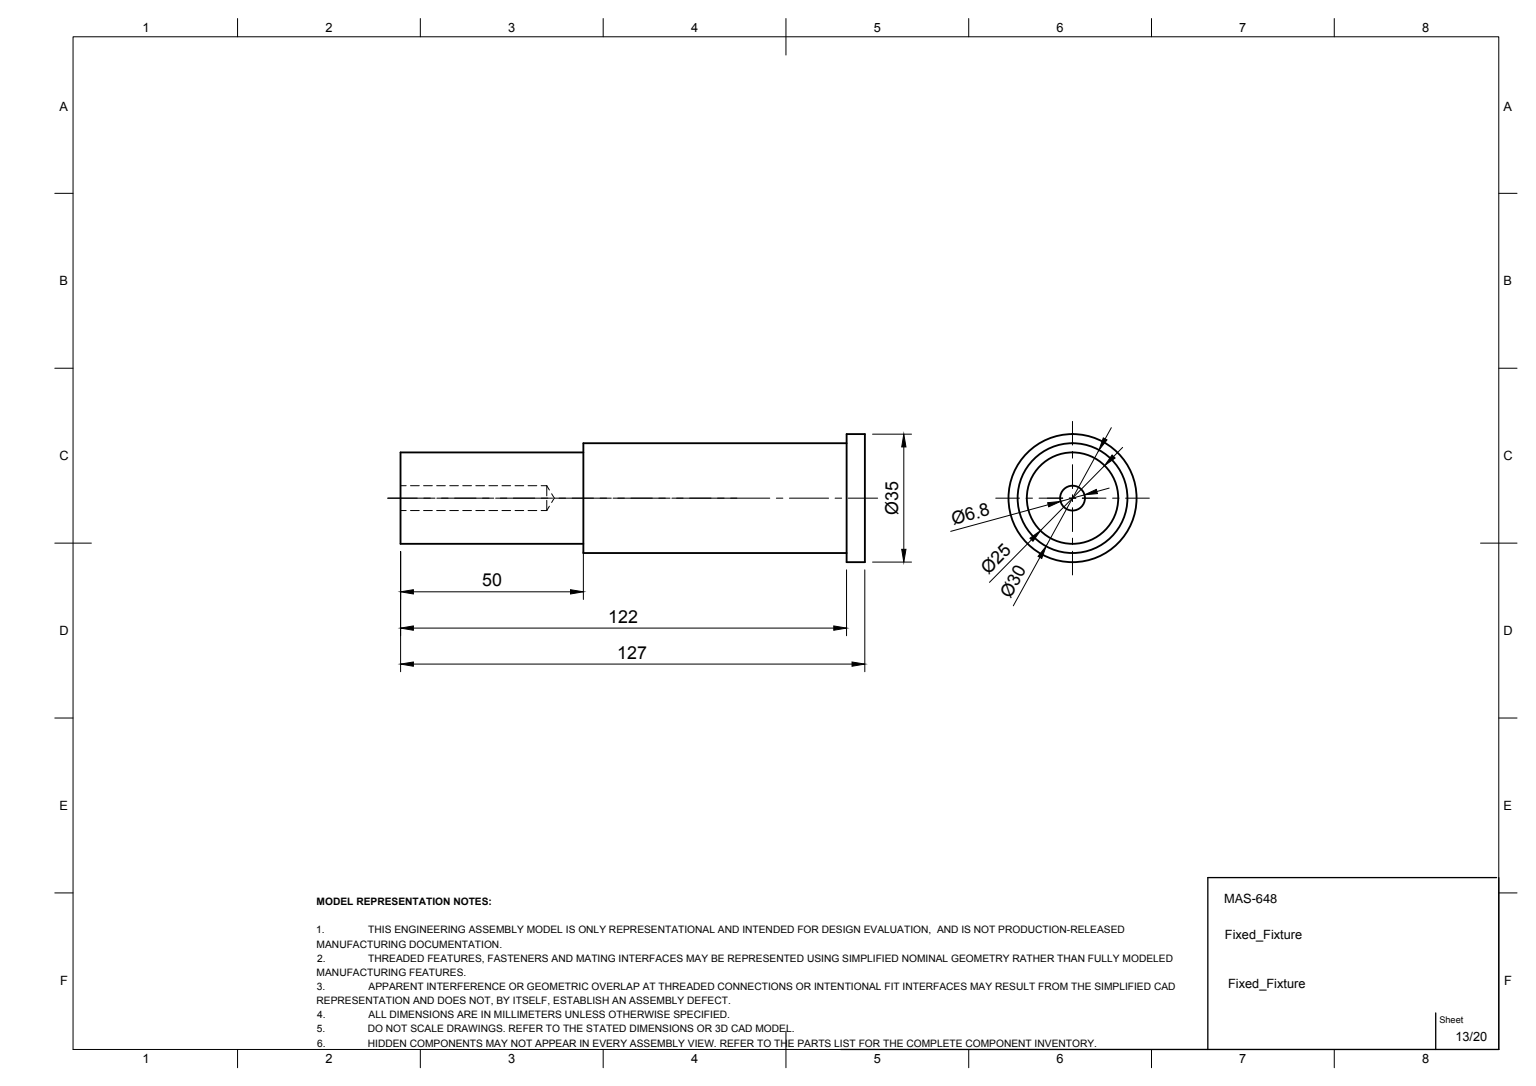
ISO-10303-21;
HEADER;
FILE_DESCRIPTION((''),'2;1');
FILE_NAME('Fixed_Fixture.step','2026-10-09T12:47:58-07:00',(''),(''),'','','');
FILE_SCHEMA (('AUTOMOTIVE_DESIGN { 1 0 10303 214 3 1 1 }'));
ENDSEC;
DATA;
#10=MECHANICAL_DESIGN_GEOMETRIC_PRESENTATION_REPRESENTATION('',(#316),#3475);
#32=CONICAL_SURFACE('',#2047,3.39999999999999,1.02974425867665) ;
#151=FACE_BOUND('',#510,.T.) ;
#152=FACE_BOUND('',#512,.T.) ;
#153=FACE_BOUND('',#514,.T.) ;
#182=CIRCLE('',#2045,3.39999999999999) ;
#183=CIRCLE('',#2046,3.39999999999999) ;
#184=CIRCLE('',#2049,12.5) ;
#185=CIRCLE('',#2050,12.5) ;
#186=CIRCLE('',#2052,15.) ;
#187=CIRCLE('',#2053,15.) ;
#188=CIRCLE('',#2055,17.5) ;
#189=CIRCLE('',#2056,17.5) ;
#265=CYLINDRICAL_SURFACE('',#2044,3.39999999999999) ;
#266=CYLINDRICAL_SURFACE('',#2048,12.5) ;
#267=CYLINDRICAL_SURFACE('',#2051,15.) ;
#268=CYLINDRICAL_SURFACE('',#2054,17.5) ;
#292=SHAPE_REPRESENTATION_RELATIONSHIP('SRR','None',#3547,#304) ;
#304=ADVANCED_BREP_SHAPE_REPRESENTATION('',(#328),#3467) ;
#316=STYLED_ITEM('',(#3628),#328) ;
#328=MANIFOLD_SOLID_BREP('Body1',#1830) ;
#379=FACE_OUTER_BOUND('',#503,.T.) ;
#380=FACE_OUTER_BOUND('',#504,.T.) ;
#381=FACE_OUTER_BOUND('',#505,.T.) ;
#382=FACE_OUTER_BOUND('',#506,.T.) ;
#383=FACE_OUTER_BOUND('',#507,.T.) ;
#384=FACE_OUTER_BOUND('',#508,.T.) ;
#385=FACE_OUTER_BOUND('',#509,.T.) ;
#386=FACE_OUTER_BOUND('',#511,.T.) ;
#387=FACE_OUTER_BOUND('',#513,.T.) ;
#503=EDGE_LOOP('',(#1388,#1389,#1390,#1391)) ;
#504=EDGE_LOOP('',(#1392,#1393,#1394)) ;
#505=EDGE_LOOP('',(#1395,#1396,#1397,#1398)) ;
#506=EDGE_LOOP('',(#1399,#1400,#1401,#1402)) ;
#507=EDGE_LOOP('',(#1403,#1404,#1405,#1406)) ;
#508=EDGE_LOOP('',(#1407)) ;
#509=EDGE_LOOP('',(#1408)) ;
#510=EDGE_LOOP('',(#1409)) ;
#511=EDGE_LOOP('',(#1410)) ;
#512=EDGE_LOOP('',(#1411)) ;
#513=EDGE_LOOP('',(#1412)) ;
#514=EDGE_LOOP('',(#1413)) ;
#664=LINE('',#3116,#783) ;
#665=LINE('',#3120,#784) ;
#666=LINE('',#3125,#785) ;
#667=LINE('',#3131,#786) ;
#668=LINE('',#3137,#787) ;
#783=VECTOR('',#2445,3.39999999999999) ;
#784=VECTOR('',#2450,3.39999999999999) ;
#785=VECTOR('',#2455,12.5) ;
#786=VECTOR('',#2462,15.) ;
#787=VECTOR('',#2469,17.5) ;
#889=VERTEX_POINT('',#3113) ;
#890=VERTEX_POINT('',#3115) ;
#891=VERTEX_POINT('',#3119) ;
#892=VERTEX_POINT('',#3122) ;
#893=VERTEX_POINT('',#3124) ;
#894=VERTEX_POINT('',#3128) ;
#895=VERTEX_POINT('',#3130) ;
#896=VERTEX_POINT('',#3134) ;
#897=VERTEX_POINT('',#3136) ;
#1066=EDGE_CURVE('',#889,#889,#182,.T.) ;
#1067=EDGE_CURVE('',#889,#890,#664,.T.) ;
#1068=EDGE_CURVE('',#890,#890,#183,.T.) ;
#1069=EDGE_CURVE('',#891,#889,#665,.T.) ;
#1070=EDGE_CURVE('',#892,#892,#184,.T.) ;
#1071=EDGE_CURVE('',#892,#893,#666,.T.) ;
#1072=EDGE_CURVE('',#893,#893,#185,.T.) ;
#1073=EDGE_CURVE('',#894,#894,#186,.T.) ;
#1074=EDGE_CURVE('',#894,#895,#667,.T.) ;
#1075=EDGE_CURVE('',#895,#895,#187,.T.) ;
#1076=EDGE_CURVE('',#896,#896,#188,.T.) ;
#1077=EDGE_CURVE('',#896,#897,#668,.T.) ;
#1078=EDGE_CURVE('',#897,#897,#189,.T.) ;
#1388=ORIENTED_EDGE('',*,*,#1066,.F.) ;
#1389=ORIENTED_EDGE('',*,*,#1067,.T.) ;
#1390=ORIENTED_EDGE('',*,*,#1068,.T.) ;
#1391=ORIENTED_EDGE('',*,*,#1067,.F.) ;
#1392=ORIENTED_EDGE('',*,*,#1069,.T.) ;
#1393=ORIENTED_EDGE('',*,*,#1066,.T.) ;
#1394=ORIENTED_EDGE('',*,*,#1069,.F.) ;
#1395=ORIENTED_EDGE('',*,*,#1070,.F.) ;
#1396=ORIENTED_EDGE('',*,*,#1071,.T.) ;
#1397=ORIENTED_EDGE('',*,*,#1072,.T.) ;
#1398=ORIENTED_EDGE('',*,*,#1071,.F.) ;
#1399=ORIENTED_EDGE('',*,*,#1073,.F.) ;
#1400=ORIENTED_EDGE('',*,*,#1074,.T.) ;
#1401=ORIENTED_EDGE('',*,*,#1075,.T.) ;
#1402=ORIENTED_EDGE('',*,*,#1074,.F.) ;
#1403=ORIENTED_EDGE('',*,*,#1076,.F.) ;
#1404=ORIENTED_EDGE('',*,*,#1077,.T.) ;
#1405=ORIENTED_EDGE('',*,*,#1078,.T.) ;
#1406=ORIENTED_EDGE('',*,*,#1077,.F.) ;
#1407=ORIENTED_EDGE('',*,*,#1078,.F.) ;
#1408=ORIENTED_EDGE('',*,*,#1076,.T.) ;
#1409=ORIENTED_EDGE('',*,*,#1075,.F.) ;
#1410=ORIENTED_EDGE('',*,*,#1073,.T.) ;
#1411=ORIENTED_EDGE('',*,*,#1072,.F.) ;
#1412=ORIENTED_EDGE('',*,*,#1070,.T.) ;
#1413=ORIENTED_EDGE('',*,*,#1068,.F.) ;
#1679=PLANE('',#2057) ;
#1680=PLANE('',#2058) ;
#1681=PLANE('',#2059) ;
#1682=PLANE('',#2060) ;
#1755=ADVANCED_FACE('',(#379),#265,.F.) ;
#1756=ADVANCED_FACE('',(#380),#32,.F.) ;
#1757=ADVANCED_FACE('',(#381),#266,.T.) ;
#1758=ADVANCED_FACE('',(#382),#267,.T.) ;
#1759=ADVANCED_FACE('',(#383),#268,.T.) ;
#1760=ADVANCED_FACE('',(#384),#1679,.T.) ;
#1761=ADVANCED_FACE('',(#385,#151),#1680,.T.) ;
#1762=ADVANCED_FACE('',(#386,#152),#1681,.T.) ;
#1763=ADVANCED_FACE('',(#387,#153),#1682,.T.) ;
#1830=CLOSED_SHELL('',(#1755,#1756,#1757,#1758,#1759,#1760,#1761,#1762,
#1763)) ;
#2043=AXIS2_PLACEMENT_3D('',#3111,#2439,#2440) ;
#2044=AXIS2_PLACEMENT_3D('',#3112,#2441,#2442) ;
#2045=AXIS2_PLACEMENT_3D('',#3114,#2443,#2444) ;
#2046=AXIS2_PLACEMENT_3D('',#3117,#2446,#2447) ;
#2047=AXIS2_PLACEMENT_3D('',#3118,#2448,#2449) ;
#2048=AXIS2_PLACEMENT_3D('',#3121,#2451,#2452) ;
#2049=AXIS2_PLACEMENT_3D('',#3123,#2453,#2454) ;
#2050=AXIS2_PLACEMENT_3D('',#3126,#2456,#2457) ;
#2051=AXIS2_PLACEMENT_3D('',#3127,#2458,#2459) ;
#2052=AXIS2_PLACEMENT_3D('',#3129,#2460,#2461) ;
#2053=AXIS2_PLACEMENT_3D('',#3132,#2463,#2464) ;
#2054=AXIS2_PLACEMENT_3D('',#3133,#2465,#2466) ;
#2055=AXIS2_PLACEMENT_3D('',#3135,#2467,#2468) ;
#2056=AXIS2_PLACEMENT_3D('',#3138,#2470,#2471) ;
#2057=AXIS2_PLACEMENT_3D('',#3139,#2472,#2473) ;
#2058=AXIS2_PLACEMENT_3D('',#3140,#2474,#2475) ;
#2059=AXIS2_PLACEMENT_3D('',#3141,#2476,#2477) ;
#2060=AXIS2_PLACEMENT_3D('',#3142,#2478,#2479) ;
#2439=DIRECTION('axis',(0.,0.,1.)) ;
#2440=DIRECTION('refdir',(1.,0.,0.)) ;
#2441=DIRECTION('center_axis',(1.,0.,0.)) ;
#2442=DIRECTION('ref_axis',(0.,0.,-1.)) ;
#2443=DIRECTION('center_axis',(1.,0.,0.)) ;
#2444=DIRECTION('ref_axis',(0.,0.,-1.)) ;
#2445=DIRECTION('',(1.,0.,0.)) ;
#2446=DIRECTION('center_axis',(1.,0.,0.)) ;
#2447=DIRECTION('ref_axis',(0.,0.,-1.)) ;
#2448=DIRECTION('center_axis',(1.,0.,0.)) ;
#2449=DIRECTION('ref_axis',(0.,0.,-1.)) ;
#2450=DIRECTION('',(0.515038074910058,-1.04972719113862E-16,0.85716730070211)) ;
#2451=DIRECTION('center_axis',(1.,0.,0.)) ;
#2452=DIRECTION('ref_axis',(0.,0.,-1.)) ;
#2453=DIRECTION('center_axis',(1.,0.,0.)) ;
#2454=DIRECTION('ref_axis',(0.,0.,-1.)) ;
#2455=DIRECTION('',(-1.,0.,0.)) ;
#2456=DIRECTION('center_axis',(1.,0.,0.)) ;
#2457=DIRECTION('ref_axis',(0.,0.,-1.)) ;
#2458=DIRECTION('center_axis',(1.,0.,0.)) ;
#2459=DIRECTION('ref_axis',(0.,0.,-1.)) ;
#2460=DIRECTION('center_axis',(1.,0.,0.)) ;
#2461=DIRECTION('ref_axis',(0.,0.,-1.)) ;
#2462=DIRECTION('',(-1.,0.,0.)) ;
#2463=DIRECTION('center_axis',(1.,0.,0.)) ;
#2464=DIRECTION('ref_axis',(0.,0.,-1.)) ;
#2465=DIRECTION('center_axis',(1.,0.,0.)) ;
#2466=DIRECTION('ref_axis',(0.,0.,-1.)) ;
#2467=DIRECTION('center_axis',(1.,0.,0.)) ;
#2468=DIRECTION('ref_axis',(0.,0.,-1.)) ;
#2469=DIRECTION('',(-1.,0.,0.)) ;
#2470=DIRECTION('center_axis',(1.,0.,0.)) ;
#2471=DIRECTION('ref_axis',(0.,0.,-1.)) ;
#2472=DIRECTION('center_axis',(-1.,0.,0.)) ;
#2473=DIRECTION('ref_axis',(0.,0.,1.)) ;
#2474=DIRECTION('center_axis',(1.,0.,0.)) ;
#2475=DIRECTION('ref_axis',(0.,0.,-1.)) ;
#2476=DIRECTION('center_axis',(1.,0.,0.)) ;
#2477=DIRECTION('ref_axis',(0.,0.,-1.)) ;
#2478=DIRECTION('center_axis',(1.,0.,0.)) ;
#2479=DIRECTION('ref_axis',(0.,0.,-1.)) ;
#3111=CARTESIAN_POINT('',(0.,0.,0.)) ;
#3112=CARTESIAN_POINT('Origin',(127.,0.,0.)) ;
#3113=CARTESIAN_POINT('',(87.,-4.16379911710099E-16,3.39999999999999)) ;
#3114=CARTESIAN_POINT('Origin',(87.,0.,0.)) ;
#3115=CARTESIAN_POINT('',(127.,-4.16379911710099E-16,3.39999999999999)) ;
#3116=CARTESIAN_POINT('',(127.,-4.16379911710099E-16,3.39999999999999)) ;
#3117=CARTESIAN_POINT('Origin',(127.,0.,0.)) ;
#3118=CARTESIAN_POINT('Origin',(87.,0.,0.)) ;
#3119=CARTESIAN_POINT('',(84.9570738953063,-1.18034773709391E-14,0.)) ;
#3120=CARTESIAN_POINT('',(87.,-4.16379911710099E-16,3.39999999999999)) ;
#3121=CARTESIAN_POINT('Origin',(127.,0.,0.)) ;
#3122=CARTESIAN_POINT('',(127.,-1.53080849893419E-15,12.5)) ;
#3123=CARTESIAN_POINT('Origin',(127.,0.,0.)) ;
#3124=CARTESIAN_POINT('',(77.,-1.53080849893419E-15,12.5)) ;
#3125=CARTESIAN_POINT('',(127.,-1.53080849893419E-15,12.5)) ;
#3126=CARTESIAN_POINT('Origin',(77.,0.,0.)) ;
#3127=CARTESIAN_POINT('Origin',(127.,0.,0.)) ;
#3128=CARTESIAN_POINT('',(77.,-1.83697019872103E-15,15.)) ;
#3129=CARTESIAN_POINT('Origin',(77.,0.,0.)) ;
#3130=CARTESIAN_POINT('',(5.00000000000002,-1.83697019872103E-15,15.)) ;
#3131=CARTESIAN_POINT('',(127.,-1.83697019872103E-15,15.)) ;
#3132=CARTESIAN_POINT('Origin',(5.,0.,0.)) ;
#3133=CARTESIAN_POINT('Origin',(127.,0.,0.)) ;
#3134=CARTESIAN_POINT('',(5.,-2.14313189850787E-15,17.5)) ;
#3135=CARTESIAN_POINT('Origin',(5.,0.,0.)) ;
#3136=CARTESIAN_POINT('',(0.,-2.14313189850787E-15,17.5)) ;
#3137=CARTESIAN_POINT('',(127.,-2.14313189850787E-15,17.5)) ;
#3138=CARTESIAN_POINT('Origin',(0.,0.,0.)) ;
#3139=CARTESIAN_POINT('Origin',(0.,0.,0.)) ;
#3140=CARTESIAN_POINT('Origin',(5.,17.5,0.)) ;
#3141=CARTESIAN_POINT('Origin',(77.,15.,0.)) ;
#3142=CARTESIAN_POINT('Origin',(127.,12.5,0.)) ;
#3449=UNCERTAINTY_MEASURE_WITH_UNIT(LENGTH_MEASURE(0.01),#3476,
'DISTANCE_ACCURACY_VALUE',
'Maximum model space distance between geometric entities at asserted c
onnectivities') ;
#3457=UNCERTAINTY_MEASURE_WITH_UNIT(LENGTH_MEASURE(0.01),#3476,
'DISTANCE_ACCURACY_VALUE',
'Maximum model space distance between geometric entities at asserted c
onnectivities') ;
#3467=(
GEOMETRIC_REPRESENTATION_CONTEXT(3)
GLOBAL_UNCERTAINTY_ASSIGNED_CONTEXT((#3449))
GLOBAL_UNIT_ASSIGNED_CONTEXT((#3476,#3478,#3479))
REPRESENTATION_CONTEXT('','3D')
) ;
#3475=(
GEOMETRIC_REPRESENTATION_CONTEXT(3)
GLOBAL_UNCERTAINTY_ASSIGNED_CONTEXT((#3457))
GLOBAL_UNIT_ASSIGNED_CONTEXT((#3476,#3478,#3479))
REPRESENTATION_CONTEXT('','3D')
) ;
#3476=(
LENGTH_UNIT()
NAMED_UNIT(*)
SI_UNIT(.MILLI.,.METRE.)
) ;
#3478=(
NAMED_UNIT(*)
PLANE_ANGLE_UNIT()
SI_UNIT($,.RADIAN.)
) ;
#3479=(
NAMED_UNIT(*)
SI_UNIT($,.STERADIAN.)
SOLID_ANGLE_UNIT()
) ;
#3489=SHAPE_DEFINITION_REPRESENTATION(#3510,#3547) ;
#3510=PRODUCT_DEFINITION_SHAPE('',$,#3565) ;
#3547=SHAPE_REPRESENTATION('',(#2043),#3467) ;
#3555=PRODUCT_DEFINITION_CONTEXT('part definition',#3608,'design') ;
#3565=PRODUCT_DEFINITION('Fixed_Fixture','Fixed_Fixture',#3582,#3555) ;
#3582=PRODUCT_DEFINITION_FORMATION('',$,#3619) ;
#3608=APPLICATION_CONTEXT(
'Core Data for Automotive Mechanical Design Process') ;
#3609=PRODUCT_CONTEXT('part definition',#3608,'mechanical') ;
#3619=PRODUCT('Fixed_Fixture',
'Fixed_Fixture',$,(#3609)) ;
#3628=PRESENTATION_STYLE_ASSIGNMENT((#3630)) ;
#3630=SURFACE_STYLE_USAGE(.BOTH.,#3632) ;
#3632=SURFACE_SIDE_STYLE('',(#3634)) ;
#3634=SURFACE_STYLE_FILL_AREA(#3636) ;
#3636=FILL_AREA_STYLE('Opaque(202,209,238)',(#3638)) ;
#3638=FILL_AREA_STYLE_COLOUR('Opaque(202,209,238)',#3640) ;
#3640=COLOUR_RGB('Opaque(202,209,238)', 0.09019608, 0.27058824, 0.51372549) ;
ENDSEC;
END-ISO-10303-21;
